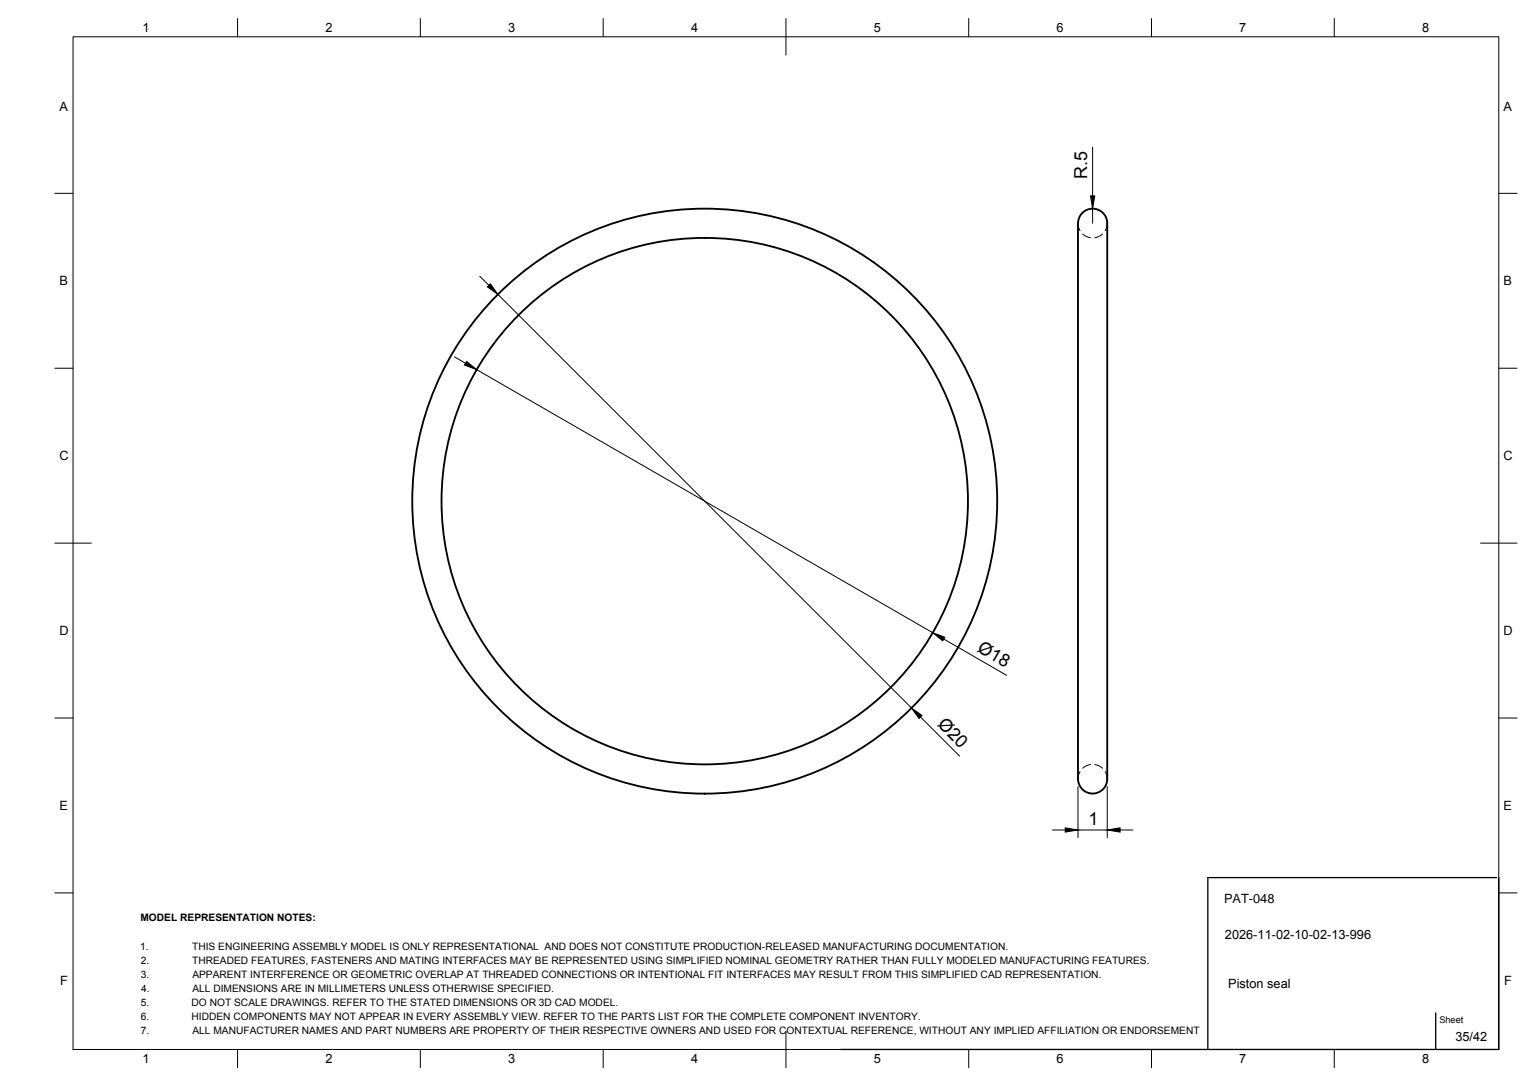
ISO-10303-21;
HEADER;
/* Generated by software containing ST-Developer
 * from STEP Tools, Inc. (www.steptools.com) 
 */

FILE_DESCRIPTION(
/* description */ ('Guided pneumatic stop gate'),
/* implementation_level */ '2;1');

FILE_NAME(
/* name */ 'Piston seal.step',
/* time_stamp */ '2026-10-27T21:43:45-07:00',
/* author */ (''),
/* organization */ (''),
/* preprocessor_version */ 'ST-DEVELOPER v20.2',
/* originating_system */ 'Autodesk Translation Framework v15.17.0.0',
/* authorisation */ '');

FILE_SCHEMA (('AUTOMOTIVE_DESIGN { 1 0 10303 214 3 1 1 }'));
ENDSEC;

DATA;
#10=MECHANICAL_DESIGN_GEOMETRIC_PRESENTATION_REPRESENTATION('',(#564),#14392);
#45=TOROIDAL_SURFACE('',#9177,0.95,0.05);
#480=SHAPE_REPRESENTATION_RELATIONSHIP('SRR','None',#14617,#522);
#522=ADVANCED_BREP_SHAPE_REPRESENTATION('',(#603),#14379);
#564=STYLED_ITEM('',(#14898),#603);
#603=MANIFOLD_SOLID_BREP('Body1',#7907);
#1486=FACE_OUTER_BOUND('',#2142,.T.);
#2142=EDGE_LOOP('',(#6802,#6803,#6804,#6805));
#3672=CIRCLE('',#9178,0.05);
#3673=CIRCLE('',#9179,0.9);
#4215=VERTEX_POINT('',#13641);
#5099=EDGE_CURVE('',#4215,#4215,#3672,.T.);
#5100=EDGE_CURVE('',#4215,#4215,#3673,.T.);
#6802=ORIENTED_EDGE('',*,*,#5099,.F.);
#6803=ORIENTED_EDGE('',*,*,#5100,.T.);
#6804=ORIENTED_EDGE('',*,*,#5099,.T.);
#6805=ORIENTED_EDGE('',*,*,#5100,.F.);
#7768=ADVANCED_FACE('',(#1486),#45,.T.);
#7907=CLOSED_SHELL('',(#7768));
#9176=AXIS2_PLACEMENT_3D('',#13639,#11378,#11379);
#9177=AXIS2_PLACEMENT_3D('',#13640,#11380,#11381);
#9178=AXIS2_PLACEMENT_3D('',#13642,#11382,#11383);
#9179=AXIS2_PLACEMENT_3D('',#13643,#11384,#11385);
#11378=DIRECTION('axis',(0.,0.,1.));
#11379=DIRECTION('refdir',(1.,0.,0.));
#11380=DIRECTION('center_axis',(0.,-1.,0.));
#11381=DIRECTION('ref_axis',(0.,0.,-1.));
#11382=DIRECTION('center_axis',(-1.,0.,-1.22464679914735E-16));
#11383=DIRECTION('ref_axis',(-1.22464679914735E-16,0.,1.));
#11384=DIRECTION('center_axis',(0.,1.,0.));
#11385=DIRECTION('ref_axis',(0.,0.,-1.));
#13639=CARTESIAN_POINT('',(0.,0.,0.));
#13640=CARTESIAN_POINT('Origin',(0.,2.95,4.5));
#13641=CARTESIAN_POINT('',(-1.10218211923262E-16,2.95,5.4));
#13642=CARTESIAN_POINT('Origin',(-1.16341445918999E-16,2.95,5.45));
#13643=CARTESIAN_POINT('Origin',(0.,2.95,4.5));
#14331=UNCERTAINTY_MEASURE_WITH_UNIT(LENGTH_MEASURE(0.001),#14393,
'DISTANCE_ACCURACY_VALUE',
'Maximum model space distance between geometric entities at asserted c
onnectivities');
#14344=UNCERTAINTY_MEASURE_WITH_UNIT(LENGTH_MEASURE(0.001),#14393,
'DISTANCE_ACCURACY_VALUE',
'Maximum model space distance between geometric entities at asserted c
onnectivities');
#14379=(
GEOMETRIC_REPRESENTATION_CONTEXT(3)
GLOBAL_UNCERTAINTY_ASSIGNED_CONTEXT((#14331))
GLOBAL_UNIT_ASSIGNED_CONTEXT((#14393,#14395,#14396))
REPRESENTATION_CONTEXT('','3D')
);
#14392=(
GEOMETRIC_REPRESENTATION_CONTEXT(3)
GLOBAL_UNCERTAINTY_ASSIGNED_CONTEXT((#14344))
GLOBAL_UNIT_ASSIGNED_CONTEXT((#14393,#14395,#14396))
REPRESENTATION_CONTEXT('','3D')
);
#14393=(
LENGTH_UNIT()
NAMED_UNIT(*)
SI_UNIT(.CENTI.,.METRE.)
);
#14395=(
NAMED_UNIT(*)
PLANE_ANGLE_UNIT()
SI_UNIT($,.RADIAN.)
);
#14396=(
NAMED_UNIT(*)
SI_UNIT($,.STERADIAN.)
SOLID_ANGLE_UNIT()
);
#14431=SHAPE_DEFINITION_REPRESENTATION(#14550,#14617);
#14550=PRODUCT_DEFINITION_SHAPE('',$,#14665);
#14617=SHAPE_REPRESENTATION('',(#9176),#14379);
#14630=PRODUCT_DEFINITION_CONTEXT('part definition',#14773,'design');
#14665=PRODUCT_DEFINITION('Piston seal','Piston seal',#14712,#14630);
#14712=PRODUCT_DEFINITION_FORMATION('',$,#14809);
#14773=APPLICATION_CONTEXT(
'Core Data for Automotive Mechanical Design Process');
#14774=PRODUCT_CONTEXT('part definition',#14773,'mechanical');
#14809=PRODUCT('Piston seal','Piston seal','Piston seal',(#14774));
#14892=COLOUR_RGB('Black',0.12,0.14,0.17);
#14893=FILL_AREA_STYLE_COLOUR('',#14892);
#14894=FILL_AREA_STYLE('',(#14893));
#14895=SURFACE_STYLE_FILL_AREA(#14894);
#14896=SURFACE_SIDE_STYLE('',(#14895));
#14897=SURFACE_STYLE_USAGE(.BOTH.,#14896);
#14898=PRESENTATION_STYLE_ASSIGNMENT((#14897));
ENDSEC;
END-ISO-10303-21;
